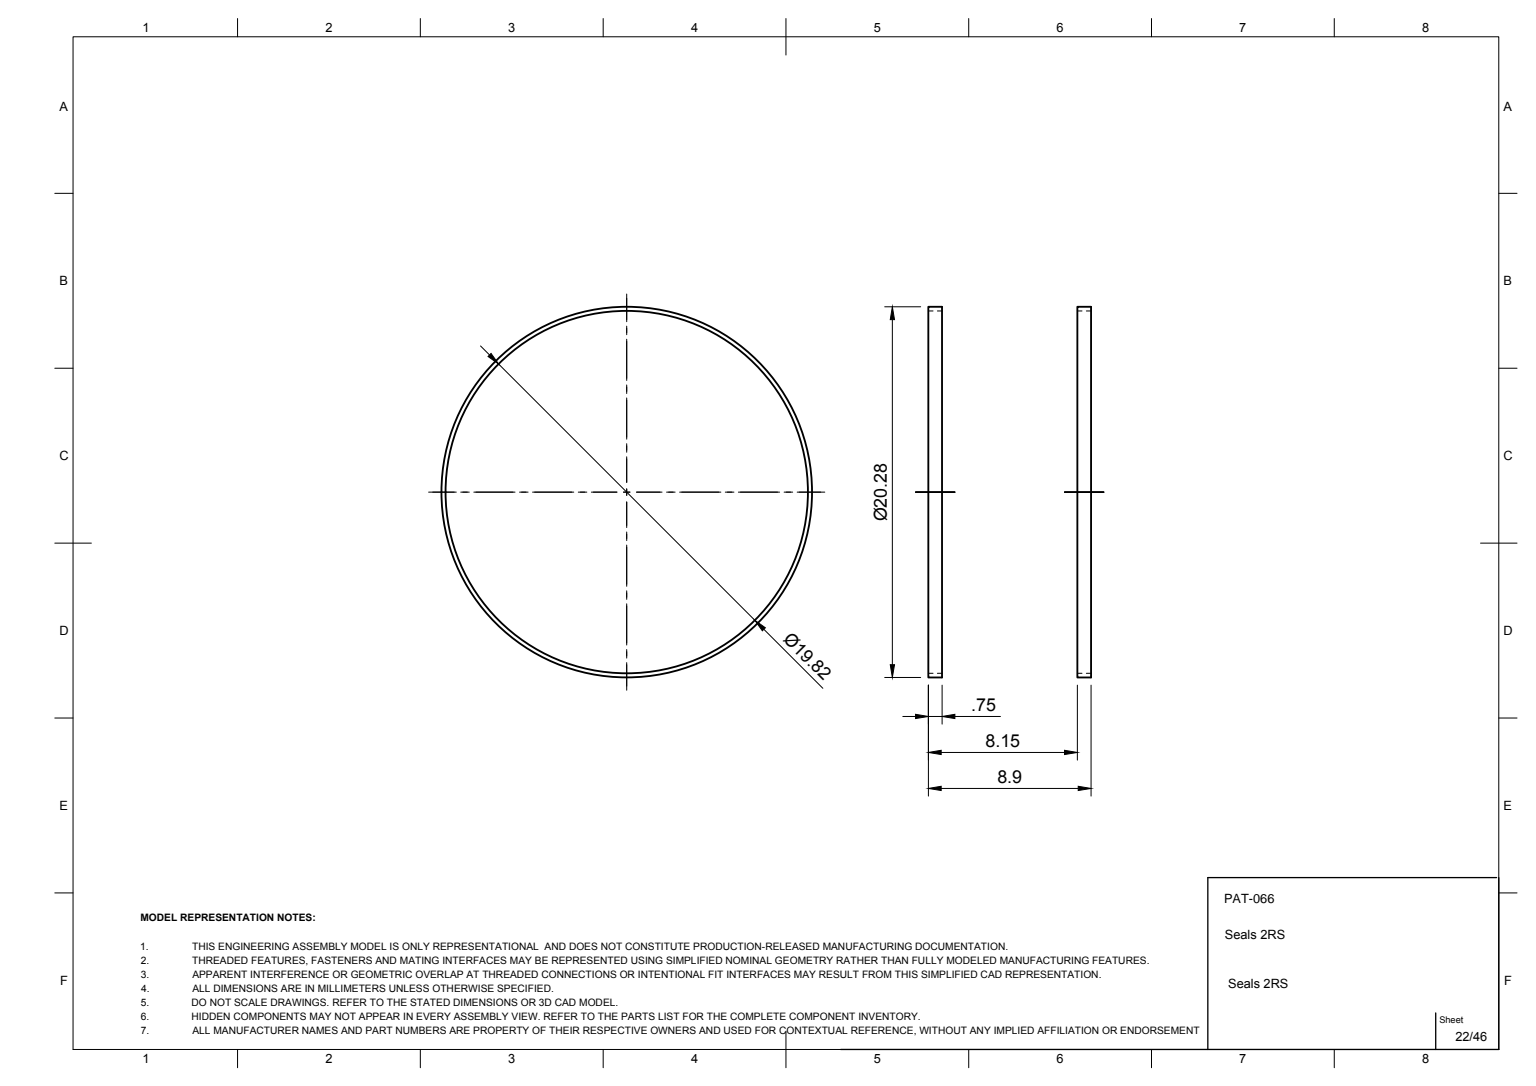
ISO-10303-21;
HEADER;
/* Generated by software containing ST-Developer
 * from STEP Tools, Inc. (www.steptools.com) 
 */

FILE_DESCRIPTION(
/* description */ ('Lever-operated bar clamp (toggle)'),
/* implementation_level */ '2;1');

FILE_NAME(
/* name */ 'Seals 2RS.step',
/* time_stamp */ '2026-10-28T03:25:02-07:00',
/* author */ (''),
/* organization */ (''),
/* preprocessor_version */ 'ST-DEVELOPER v20.2',
/* originating_system */ 'Autodesk Translation Framework v15.17.0.0',
/* authorisation */ '');

FILE_SCHEMA (('AUTOMOTIVE_DESIGN { 1 0 10303 214 3 1 1 }'));
ENDSEC;

DATA;
#10=MECHANICAL_DESIGN_GEOMETRIC_PRESENTATION_REPRESENTATION('',(#433,#434),#12413);
#350=SHAPE_REPRESENTATION_RELATIONSHIP('SRR','None',#12590,#388);
#388=ADVANCED_BREP_SHAPE_REPRESENTATION('',(#479,#480),#12387);
#433=STYLED_ITEM('',(#12869),#479);
#434=STYLED_ITEM('',(#12869),#480);
#479=MANIFOLD_SOLID_BREP('Body1',#6593);
#480=MANIFOLD_SOLID_BREP('Body2',#6594);
#593=FACE_BOUND('',#1582,.T.);
#594=FACE_BOUND('',#1585,.T.);
#595=FACE_BOUND('',#1588,.T.);
#596=FACE_BOUND('',#1591,.T.);
#752=PLANE('',#7440);
#753=PLANE('',#7445);
#754=PLANE('',#7448);
#755=PLANE('',#7453);
#1082=FACE_OUTER_BOUND('',#1581,.T.);
#1083=FACE_OUTER_BOUND('',#1583,.T.);
#1084=FACE_OUTER_BOUND('',#1584,.T.);
#1085=FACE_OUTER_BOUND('',#1586,.T.);
#1086=FACE_OUTER_BOUND('',#1587,.T.);
#1087=FACE_OUTER_BOUND('',#1589,.T.);
#1088=FACE_OUTER_BOUND('',#1590,.T.);
#1089=FACE_OUTER_BOUND('',#1592,.T.);
#1581=EDGE_LOOP('',(#5233));
#1582=EDGE_LOOP('',(#5234));
#1583=EDGE_LOOP('',(#5235,#5236,#5237,#5238));
#1584=EDGE_LOOP('',(#5239));
#1585=EDGE_LOOP('',(#5240));
#1586=EDGE_LOOP('',(#5241,#5242,#5243,#5244));
#1587=EDGE_LOOP('',(#5245));
#1588=EDGE_LOOP('',(#5246));
#1589=EDGE_LOOP('',(#5247,#5248,#5249,#5250));
#1590=EDGE_LOOP('',(#5251));
#1591=EDGE_LOOP('',(#5252));
#1592=EDGE_LOOP('',(#5253,#5254,#5255,#5256));
#2052=LINE('',#11290,#2493);
#2053=LINE('',#11295,#2494);
#2054=LINE('',#11304,#2495);
#2055=LINE('',#11309,#2496);
#2493=VECTOR('',#8907,1.013815);
#2494=VECTOR('',#8914,0.991185);
#2495=VECTOR('',#8925,1.013815);
#2496=VECTOR('',#8932,0.991185);
#2920=CIRCLE('',#7441,1.013815);
#2921=CIRCLE('',#7442,0.991185);
#2922=CIRCLE('',#7444,1.013815);
#2923=CIRCLE('',#7446,0.991185);
#2924=CIRCLE('',#7449,1.013815);
#2925=CIRCLE('',#7450,0.991185);
#2926=CIRCLE('',#7452,1.013815);
#2927=CIRCLE('',#7454,0.991185);
#3353=VERTEX_POINT('',#11283);
#3354=VERTEX_POINT('',#11285);
#3355=VERTEX_POINT('',#11288);
#3356=VERTEX_POINT('',#11292);
#3357=VERTEX_POINT('',#11297);
#3358=VERTEX_POINT('',#11299);
#3359=VERTEX_POINT('',#11302);
#3360=VERTEX_POINT('',#11306);
#4021=EDGE_CURVE('',#3353,#3353,#2920,.T.);
#4022=EDGE_CURVE('',#3354,#3354,#2921,.T.);
#4023=EDGE_CURVE('',#3355,#3355,#2922,.T.);
#4024=EDGE_CURVE('',#3355,#3353,#2052,.T.);
#4025=EDGE_CURVE('',#3356,#3356,#2923,.T.);
#4026=EDGE_CURVE('',#3356,#3354,#2053,.T.);
#4027=EDGE_CURVE('',#3357,#3357,#2924,.T.);
#4028=EDGE_CURVE('',#3358,#3358,#2925,.T.);
#4029=EDGE_CURVE('',#3359,#3359,#2926,.T.);
#4030=EDGE_CURVE('',#3359,#3357,#2054,.T.);
#4031=EDGE_CURVE('',#3360,#3360,#2927,.T.);
#4032=EDGE_CURVE('',#3360,#3358,#2055,.T.);
#5233=ORIENTED_EDGE('',*,*,#4021,.F.);
#5234=ORIENTED_EDGE('',*,*,#4022,.T.);
#5235=ORIENTED_EDGE('',*,*,#4023,.F.);
#5236=ORIENTED_EDGE('',*,*,#4024,.T.);
#5237=ORIENTED_EDGE('',*,*,#4021,.T.);
#5238=ORIENTED_EDGE('',*,*,#4024,.F.);
#5239=ORIENTED_EDGE('',*,*,#4023,.T.);
#5240=ORIENTED_EDGE('',*,*,#4025,.F.);
#5241=ORIENTED_EDGE('',*,*,#4025,.T.);
#5242=ORIENTED_EDGE('',*,*,#4026,.T.);
#5243=ORIENTED_EDGE('',*,*,#4022,.F.);
#5244=ORIENTED_EDGE('',*,*,#4026,.F.);
#5245=ORIENTED_EDGE('',*,*,#4027,.F.);
#5246=ORIENTED_EDGE('',*,*,#4028,.T.);
#5247=ORIENTED_EDGE('',*,*,#4029,.F.);
#5248=ORIENTED_EDGE('',*,*,#4030,.T.);
#5249=ORIENTED_EDGE('',*,*,#4027,.T.);
#5250=ORIENTED_EDGE('',*,*,#4030,.F.);
#5251=ORIENTED_EDGE('',*,*,#4029,.T.);
#5252=ORIENTED_EDGE('',*,*,#4031,.F.);
#5253=ORIENTED_EDGE('',*,*,#4031,.T.);
#5254=ORIENTED_EDGE('',*,*,#4032,.T.);
#5255=ORIENTED_EDGE('',*,*,#4028,.F.);
#5256=ORIENTED_EDGE('',*,*,#4032,.F.);
#6101=CYLINDRICAL_SURFACE('',#7443,1.013815);
#6102=CYLINDRICAL_SURFACE('',#7447,0.991185);
#6103=CYLINDRICAL_SURFACE('',#7451,1.013815);
#6104=CYLINDRICAL_SURFACE('',#7455,0.991185);
#6357=ADVANCED_FACE('',(#1082,#593),#752,.T.);
#6358=ADVANCED_FACE('',(#1083),#6101,.T.);
#6359=ADVANCED_FACE('',(#1084,#594),#753,.T.);
#6360=ADVANCED_FACE('',(#1085),#6102,.F.);
#6361=ADVANCED_FACE('',(#1086,#595),#754,.T.);
#6362=ADVANCED_FACE('',(#1087),#6103,.T.);
#6363=ADVANCED_FACE('',(#1088,#596),#755,.T.);
#6364=ADVANCED_FACE('',(#1089),#6104,.F.);
#6593=CLOSED_SHELL('',(#6357,#6358,#6359,#6360));
#6594=CLOSED_SHELL('',(#6361,#6362,#6363,#6364));
#7439=AXIS2_PLACEMENT_3D('',#11281,#8895,#8896);
#7440=AXIS2_PLACEMENT_3D('',#11282,#8897,#8898);
#7441=AXIS2_PLACEMENT_3D('',#11284,#8899,#8900);
#7442=AXIS2_PLACEMENT_3D('',#11286,#8901,#8902);
#7443=AXIS2_PLACEMENT_3D('',#11287,#8903,#8904);
#7444=AXIS2_PLACEMENT_3D('',#11289,#8905,#8906);
#7445=AXIS2_PLACEMENT_3D('',#11291,#8908,#8909);
#7446=AXIS2_PLACEMENT_3D('',#11293,#8910,#8911);
#7447=AXIS2_PLACEMENT_3D('',#11294,#8912,#8913);
#7448=AXIS2_PLACEMENT_3D('',#11296,#8915,#8916);
#7449=AXIS2_PLACEMENT_3D('',#11298,#8917,#8918);
#7450=AXIS2_PLACEMENT_3D('',#11300,#8919,#8920);
#7451=AXIS2_PLACEMENT_3D('',#11301,#8921,#8922);
#7452=AXIS2_PLACEMENT_3D('',#11303,#8923,#8924);
#7453=AXIS2_PLACEMENT_3D('',#11305,#8926,#8927);
#7454=AXIS2_PLACEMENT_3D('',#11307,#8928,#8929);
#7455=AXIS2_PLACEMENT_3D('',#11308,#8930,#8931);
#8895=DIRECTION('axis',(0.,0.,1.));
#8896=DIRECTION('refdir',(1.,0.,0.));
#8897=DIRECTION('center_axis',(0.,1.,0.));
#8898=DIRECTION('ref_axis',(0.,0.,1.));
#8899=DIRECTION('center_axis',(0.,-1.,0.));
#8900=DIRECTION('ref_axis',(1.,0.,0.));
#8901=DIRECTION('center_axis',(0.,-1.,0.));
#8902=DIRECTION('ref_axis',(1.,0.,0.));
#8903=DIRECTION('center_axis',(0.,-1.,0.));
#8904=DIRECTION('ref_axis',(1.,0.,0.));
#8905=DIRECTION('center_axis',(0.,-1.,0.));
#8906=DIRECTION('ref_axis',(1.,0.,0.));
#8907=DIRECTION('',(0.,1.,0.));
#8908=DIRECTION('center_axis',(0.,-1.,0.));
#8909=DIRECTION('ref_axis',(0.,0.,-1.));
#8910=DIRECTION('center_axis',(0.,-1.,0.));
#8911=DIRECTION('ref_axis',(1.,0.,0.));
#8912=DIRECTION('center_axis',(0.,-1.,0.));
#8913=DIRECTION('ref_axis',(1.,0.,0.));
#8914=DIRECTION('',(0.,1.,0.));
#8915=DIRECTION('center_axis',(0.,1.,0.));
#8916=DIRECTION('ref_axis',(0.,0.,1.));
#8917=DIRECTION('center_axis',(0.,-1.,0.));
#8918=DIRECTION('ref_axis',(1.,0.,0.));
#8919=DIRECTION('center_axis',(0.,-1.,0.));
#8920=DIRECTION('ref_axis',(1.,0.,0.));
#8921=DIRECTION('center_axis',(0.,-1.,0.));
#8922=DIRECTION('ref_axis',(1.,0.,0.));
#8923=DIRECTION('center_axis',(0.,-1.,0.));
#8924=DIRECTION('ref_axis',(1.,0.,0.));
#8925=DIRECTION('',(0.,1.,0.));
#8926=DIRECTION('center_axis',(0.,-1.,0.));
#8927=DIRECTION('ref_axis',(0.,0.,-1.));
#8928=DIRECTION('center_axis',(0.,-1.,0.));
#8929=DIRECTION('ref_axis',(1.,0.,0.));
#8930=DIRECTION('center_axis',(0.,-1.,0.));
#8931=DIRECTION('ref_axis',(1.,0.,0.));
#8932=DIRECTION('',(0.,1.,0.));
#11281=CARTESIAN_POINT('',(0.,0.,0.));
#11282=CARTESIAN_POINT('Origin',(1.013815,0.445,0.));
#11283=CARTESIAN_POINT('',(-1.013815,0.445,-1.24156529467757E-16));
#11284=CARTESIAN_POINT('Origin',(0.,0.445,0.));
#11285=CARTESIAN_POINT('',(-0.991185,0.445,-1.21385153761287E-16));
#11286=CARTESIAN_POINT('Origin',(0.,0.445,0.));
#11287=CARTESIAN_POINT('Origin',(0.,0.4075,0.));
#11288=CARTESIAN_POINT('',(-1.013815,0.37,-1.24156529467757E-16));
#11289=CARTESIAN_POINT('Origin',(0.,0.37,0.));
#11290=CARTESIAN_POINT('',(-1.013815,0.4075,-1.24156529467757E-16));
#11291=CARTESIAN_POINT('Origin',(0.991185,0.37,0.));
#11292=CARTESIAN_POINT('',(-0.991185,0.37,-1.21385153761287E-16));
#11293=CARTESIAN_POINT('Origin',(0.,0.37,0.));
#11294=CARTESIAN_POINT('Origin',(0.,0.4075,0.));
#11295=CARTESIAN_POINT('',(-0.991185,0.4075,-1.21385153761287E-16));
#11296=CARTESIAN_POINT('Origin',(1.013815,-0.37,0.));
#11297=CARTESIAN_POINT('',(-1.013815,-0.37,-1.24156529467757E-16));
#11298=CARTESIAN_POINT('Origin',(0.,-0.37,0.));
#11299=CARTESIAN_POINT('',(-0.991185,-0.37,-1.21385153761287E-16));
#11300=CARTESIAN_POINT('Origin',(0.,-0.37,0.));
#11301=CARTESIAN_POINT('Origin',(0.,-0.4075,0.));
#11302=CARTESIAN_POINT('',(-1.013815,-0.445,-1.24156529467757E-16));
#11303=CARTESIAN_POINT('Origin',(0.,-0.445,0.));
#11304=CARTESIAN_POINT('',(-1.013815,-0.4075,-1.24156529467757E-16));
#11305=CARTESIAN_POINT('Origin',(0.991185,-0.445,0.));
#11306=CARTESIAN_POINT('',(-0.991185,-0.445,-1.21385153761287E-16));
#11307=CARTESIAN_POINT('Origin',(0.,-0.445,0.));
#11308=CARTESIAN_POINT('Origin',(0.,-0.4075,0.));
#11309=CARTESIAN_POINT('',(-0.991185,-0.4075,-1.21385153761287E-16));
#12341=UNCERTAINTY_MEASURE_WITH_UNIT(LENGTH_MEASURE(0.001),#12414,
'DISTANCE_ACCURACY_VALUE',
'Maximum model space distance between geometric entities at asserted c
onnectivities');
#12367=UNCERTAINTY_MEASURE_WITH_UNIT(LENGTH_MEASURE(0.001),#12414,
'DISTANCE_ACCURACY_VALUE',
'Maximum model space distance between geometric entities at asserted c
onnectivities');
#12387=(
GEOMETRIC_REPRESENTATION_CONTEXT(3)
GLOBAL_UNCERTAINTY_ASSIGNED_CONTEXT((#12341))
GLOBAL_UNIT_ASSIGNED_CONTEXT((#12414,#12416,#12417))
REPRESENTATION_CONTEXT('','3D')
);
#12413=(
GEOMETRIC_REPRESENTATION_CONTEXT(3)
GLOBAL_UNCERTAINTY_ASSIGNED_CONTEXT((#12367))
GLOBAL_UNIT_ASSIGNED_CONTEXT((#12414,#12416,#12417))
REPRESENTATION_CONTEXT('','3D')
);
#12414=(
LENGTH_UNIT()
NAMED_UNIT(*)
SI_UNIT(.CENTI.,.METRE.)
);
#12416=(
NAMED_UNIT(*)
PLANE_ANGLE_UNIT()
SI_UNIT($,.RADIAN.)
);
#12417=(
NAMED_UNIT(*)
SI_UNIT($,.STERADIAN.)
SOLID_ANGLE_UNIT()
);
#12437=SHAPE_DEFINITION_REPRESENTATION(#12482,#12590);
#12482=PRODUCT_DEFINITION_SHAPE('',$,#12636);
#12590=SHAPE_REPRESENTATION('',(#7439),#12387);
#12616=PRODUCT_DEFINITION_CONTEXT('part definition',#12753,'design');
#12636=PRODUCT_DEFINITION('Seals 2RS','Seals 2RS',#12681,#12616);
#12681=PRODUCT_DEFINITION_FORMATION('',$,#12774);
#12753=APPLICATION_CONTEXT(
'Core Data for Automotive Mechanical Design Process');
#12754=PRODUCT_CONTEXT('part definition',#12753,'mechanical');
#12774=PRODUCT('Seals 2RS','Seals 2RS','Seals 2RS',(#12754));
#12863=COLOUR_RGB('Grey',0.48,0.52,0.57);
#12864=FILL_AREA_STYLE_COLOUR('',#12863);
#12865=FILL_AREA_STYLE('',(#12864));
#12866=SURFACE_STYLE_FILL_AREA(#12865);
#12867=SURFACE_SIDE_STYLE('',(#12866));
#12868=SURFACE_STYLE_USAGE(.BOTH.,#12867);
#12869=PRESENTATION_STYLE_ASSIGNMENT((#12868));
ENDSEC;
END-ISO-10303-21;
